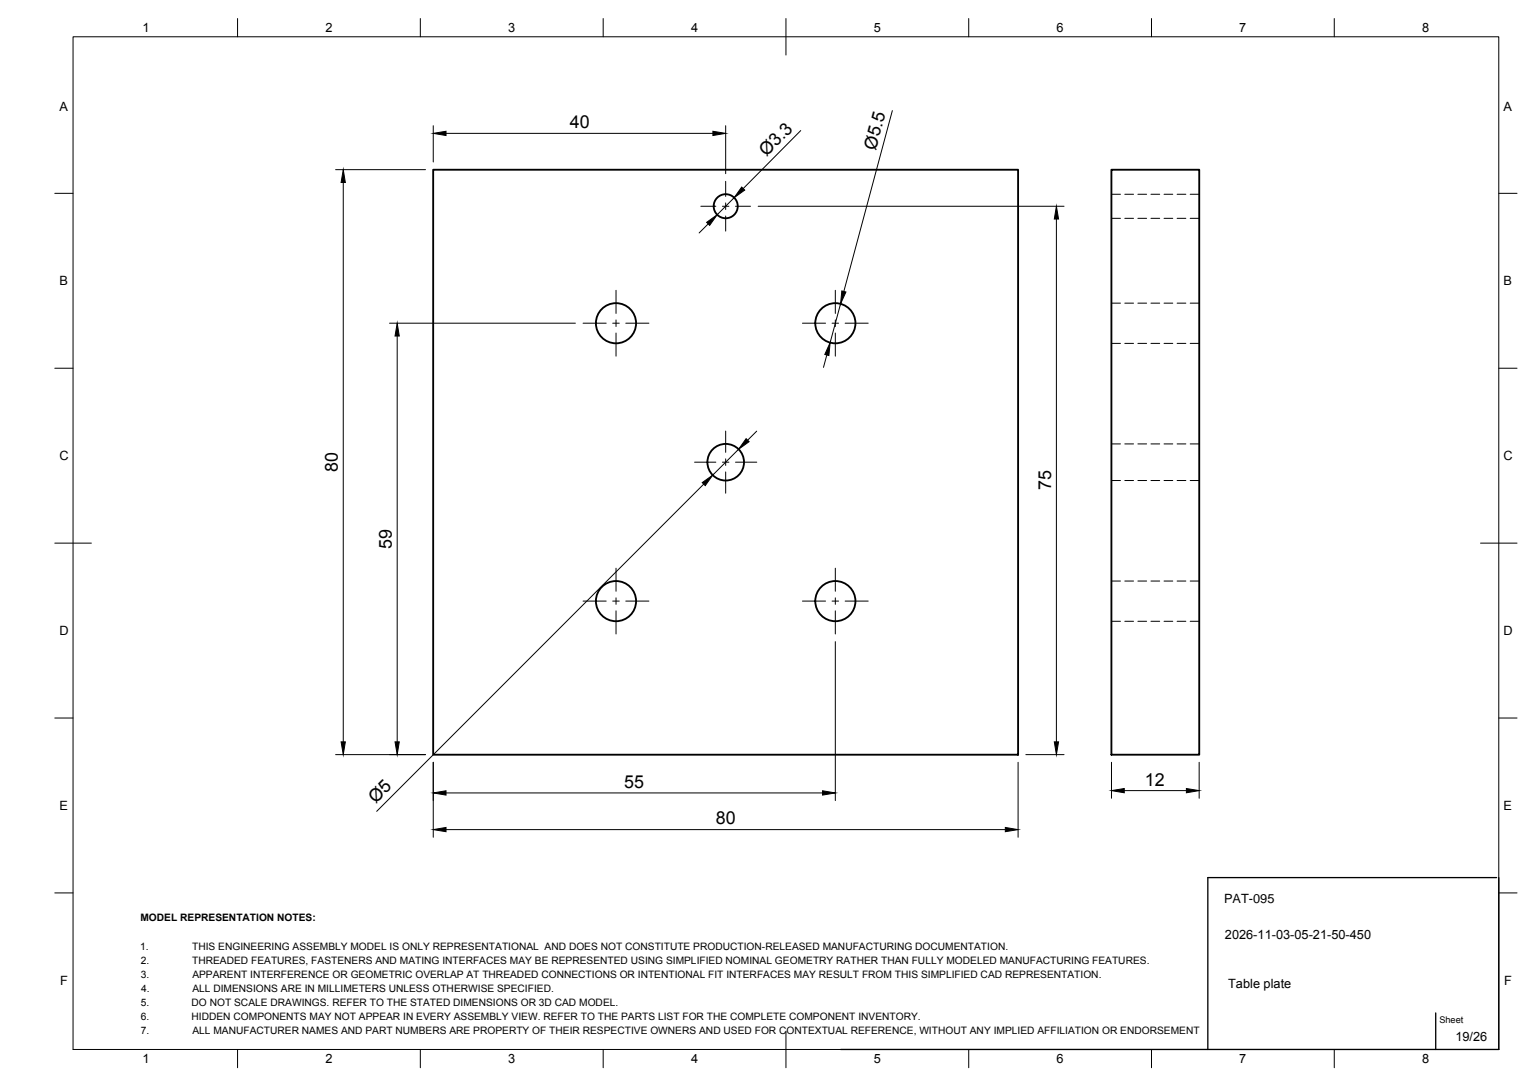
ISO-10303-21;
HEADER;
/* Generated by software containing ST-Developer
 * from STEP Tools, Inc. (www.steptools.com) 
 */

FILE_DESCRIPTION(
/* description */ ('Single-Axis Profile-Rail Linear Slide'),
/* implementation_level */ '2;1');

FILE_NAME(
/* name */ 'Table plate.step',
/* time_stamp */ '2026-10-27T10:47:43-07:00',
/* author */ (''),
/* organization */ (''),
/* preprocessor_version */ 'ST-DEVELOPER v20.2',
/* originating_system */ 'Autodesk Translation Framework v15.17.0.0',
/* authorisation */ '');

FILE_SCHEMA (('AUTOMOTIVE_DESIGN { 1 0 10303 214 3 1 1 }'));
ENDSEC;

DATA;
#10=MECHANICAL_DESIGN_GEOMETRIC_PRESENTATION_REPRESENTATION('',(#344),#14478);
#290=SHAPE_REPRESENTATION_RELATIONSHIP('SRR','None',#14621,#317);
#317=ADVANCED_BREP_SHAPE_REPRESENTATION('',(#369),#14465);
#344=STYLED_ITEM('',(#14824),#369);
#369=MANIFOLD_SOLID_BREP('Body1',#8606);
#439=FACE_BOUND('',#1690,.T.);
#440=FACE_BOUND('',#1691,.T.);
#441=FACE_BOUND('',#1692,.T.);
#442=FACE_BOUND('',#1693,.T.);
#443=FACE_BOUND('',#1694,.T.);
#444=FACE_BOUND('',#1695,.T.);
#445=FACE_BOUND('',#1697,.T.);
#446=FACE_BOUND('',#1698,.T.);
#447=FACE_BOUND('',#1699,.T.);
#448=FACE_BOUND('',#1700,.T.);
#449=FACE_BOUND('',#1701,.T.);
#450=FACE_BOUND('',#1702,.T.);
#747=PLANE('',#9365);
#748=PLANE('',#9366);
#749=PLANE('',#9367);
#750=PLANE('',#9368);
#751=PLANE('',#9369);
#752=PLANE('',#9370);
#1163=FACE_OUTER_BOUND('',#1679,.T.);
#1164=FACE_OUTER_BOUND('',#1680,.T.);
#1165=FACE_OUTER_BOUND('',#1681,.T.);
#1166=FACE_OUTER_BOUND('',#1682,.T.);
#1167=FACE_OUTER_BOUND('',#1683,.T.);
#1168=FACE_OUTER_BOUND('',#1684,.T.);
#1169=FACE_OUTER_BOUND('',#1685,.T.);
#1170=FACE_OUTER_BOUND('',#1686,.T.);
#1171=FACE_OUTER_BOUND('',#1687,.T.);
#1172=FACE_OUTER_BOUND('',#1688,.T.);
#1173=FACE_OUTER_BOUND('',#1689,.T.);
#1174=FACE_OUTER_BOUND('',#1696,.T.);
#1679=EDGE_LOOP('',(#7481,#7482,#7483,#7484));
#1680=EDGE_LOOP('',(#7485,#7486,#7487,#7488));
#1681=EDGE_LOOP('',(#7489,#7490,#7491,#7492));
#1682=EDGE_LOOP('',(#7493,#7494,#7495,#7496));
#1683=EDGE_LOOP('',(#7497,#7498,#7499,#7500));
#1684=EDGE_LOOP('',(#7501,#7502,#7503,#7504));
#1685=EDGE_LOOP('',(#7505,#7506,#7507,#7508));
#1686=EDGE_LOOP('',(#7509,#7510,#7511,#7512));
#1687=EDGE_LOOP('',(#7513,#7514,#7515,#7516));
#1688=EDGE_LOOP('',(#7517,#7518,#7519,#7520));
#1689=EDGE_LOOP('',(#7521,#7522,#7523,#7524));
#1690=EDGE_LOOP('',(#7525));
#1691=EDGE_LOOP('',(#7526));
#1692=EDGE_LOOP('',(#7527));
#1693=EDGE_LOOP('',(#7528));
#1694=EDGE_LOOP('',(#7529));
#1695=EDGE_LOOP('',(#7530));
#1696=EDGE_LOOP('',(#7531,#7532,#7533,#7534));
#1697=EDGE_LOOP('',(#7535));
#1698=EDGE_LOOP('',(#7536));
#1699=EDGE_LOOP('',(#7537));
#1700=EDGE_LOOP('',(#7538));
#1701=EDGE_LOOP('',(#7539));
#1702=EDGE_LOOP('',(#7540));
#2588=LINE('',#13730,#3559);
#2589=LINE('',#13736,#3560);
#2590=LINE('',#13742,#3561);
#2591=LINE('',#13748,#3562);
#2592=LINE('',#13754,#3563);
#2593=LINE('',#13760,#3564);
#2594=LINE('',#13765,#3565);
#2595=LINE('',#13767,#3566);
#2596=LINE('',#13769,#3567);
#2597=LINE('',#13770,#3568);
#2598=LINE('',#13773,#3569);
#2599=LINE('',#13775,#3570);
#2600=LINE('',#13776,#3571);
#2601=LINE('',#13779,#3572);
#2602=LINE('',#13781,#3573);
#2603=LINE('',#13782,#3574);
#2604=LINE('',#13784,#3575);
#2605=LINE('',#13785,#3576);
#3559=VECTOR('',#11229,0.164999999999999);
#3560=VECTOR('',#11236,0.25);
#3561=VECTOR('',#11243,0.275);
#3562=VECTOR('',#11250,0.275);
#3563=VECTOR('',#11257,0.275);
#3564=VECTOR('',#11264,0.275);
#3565=VECTOR('',#11269,1.);
#3566=VECTOR('',#11270,1.);
#3567=VECTOR('',#11271,1.);
#3568=VECTOR('',#11272,1.);
#3569=VECTOR('',#11275,1.);
#3570=VECTOR('',#11276,1.);
#3571=VECTOR('',#11277,1.);
#3572=VECTOR('',#11280,1.);
#3573=VECTOR('',#11281,1.);
#3574=VECTOR('',#11282,1.);
#3575=VECTOR('',#11285,1.);
#3576=VECTOR('',#11286,1.);
#3866=CIRCLE('',#9348,0.164999999999999);
#3867=CIRCLE('',#9349,0.164999999999999);
#3868=CIRCLE('',#9351,0.25);
#3869=CIRCLE('',#9352,0.25);
#3870=CIRCLE('',#9354,0.275);
#3871=CIRCLE('',#9355,0.275);
#3872=CIRCLE('',#9357,0.275);
#3873=CIRCLE('',#9358,0.275);
#3874=CIRCLE('',#9360,0.275);
#3875=CIRCLE('',#9361,0.275);
#3876=CIRCLE('',#9363,0.275);
#3877=CIRCLE('',#9364,0.275);
#4492=VERTEX_POINT('',#13727);
#4493=VERTEX_POINT('',#13729);
#4494=VERTEX_POINT('',#13733);
#4495=VERTEX_POINT('',#13735);
#4496=VERTEX_POINT('',#13739);
#4497=VERTEX_POINT('',#13741);
#4498=VERTEX_POINT('',#13745);
#4499=VERTEX_POINT('',#13747);
#4500=VERTEX_POINT('',#13751);
#4501=VERTEX_POINT('',#13753);
#4502=VERTEX_POINT('',#13757);
#4503=VERTEX_POINT('',#13759);
#4504=VERTEX_POINT('',#13763);
#4505=VERTEX_POINT('',#13764);
#4506=VERTEX_POINT('',#13766);
#4507=VERTEX_POINT('',#13768);
#4508=VERTEX_POINT('',#13772);
#4509=VERTEX_POINT('',#13774);
#4510=VERTEX_POINT('',#13778);
#4511=VERTEX_POINT('',#13780);
#5518=EDGE_CURVE('',#4492,#4492,#3866,.T.);
#5519=EDGE_CURVE('',#4492,#4493,#2588,.T.);
#5520=EDGE_CURVE('',#4493,#4493,#3867,.T.);
#5521=EDGE_CURVE('',#4494,#4494,#3868,.T.);
#5522=EDGE_CURVE('',#4494,#4495,#2589,.T.);
#5523=EDGE_CURVE('',#4495,#4495,#3869,.T.);
#5524=EDGE_CURVE('',#4496,#4496,#3870,.T.);
#5525=EDGE_CURVE('',#4496,#4497,#2590,.T.);
#5526=EDGE_CURVE('',#4497,#4497,#3871,.T.);
#5527=EDGE_CURVE('',#4498,#4498,#3872,.T.);
#5528=EDGE_CURVE('',#4498,#4499,#2591,.T.);
#5529=EDGE_CURVE('',#4499,#4499,#3873,.T.);
#5530=EDGE_CURVE('',#4500,#4500,#3874,.T.);
#5531=EDGE_CURVE('',#4500,#4501,#2592,.T.);
#5532=EDGE_CURVE('',#4501,#4501,#3875,.T.);
#5533=EDGE_CURVE('',#4502,#4502,#3876,.T.);
#5534=EDGE_CURVE('',#4502,#4503,#2593,.T.);
#5535=EDGE_CURVE('',#4503,#4503,#3877,.T.);
#5536=EDGE_CURVE('',#4504,#4505,#2594,.T.);
#5537=EDGE_CURVE('',#4505,#4506,#2595,.T.);
#5538=EDGE_CURVE('',#4507,#4506,#2596,.T.);
#5539=EDGE_CURVE('',#4504,#4507,#2597,.T.);
#5540=EDGE_CURVE('',#4508,#4504,#2598,.T.);
#5541=EDGE_CURVE('',#4509,#4507,#2599,.T.);
#5542=EDGE_CURVE('',#4508,#4509,#2600,.T.);
#5543=EDGE_CURVE('',#4510,#4508,#2601,.T.);
#5544=EDGE_CURVE('',#4511,#4509,#2602,.T.);
#5545=EDGE_CURVE('',#4510,#4511,#2603,.T.);
#5546=EDGE_CURVE('',#4505,#4510,#2604,.T.);
#5547=EDGE_CURVE('',#4506,#4511,#2605,.T.);
#7481=ORIENTED_EDGE('',*,*,#5518,.F.);
#7482=ORIENTED_EDGE('',*,*,#5519,.T.);
#7483=ORIENTED_EDGE('',*,*,#5520,.F.);
#7484=ORIENTED_EDGE('',*,*,#5519,.F.);
#7485=ORIENTED_EDGE('',*,*,#5521,.F.);
#7486=ORIENTED_EDGE('',*,*,#5522,.T.);
#7487=ORIENTED_EDGE('',*,*,#5523,.F.);
#7488=ORIENTED_EDGE('',*,*,#5522,.F.);
#7489=ORIENTED_EDGE('',*,*,#5524,.F.);
#7490=ORIENTED_EDGE('',*,*,#5525,.T.);
#7491=ORIENTED_EDGE('',*,*,#5526,.F.);
#7492=ORIENTED_EDGE('',*,*,#5525,.F.);
#7493=ORIENTED_EDGE('',*,*,#5527,.F.);
#7494=ORIENTED_EDGE('',*,*,#5528,.T.);
#7495=ORIENTED_EDGE('',*,*,#5529,.F.);
#7496=ORIENTED_EDGE('',*,*,#5528,.F.);
#7497=ORIENTED_EDGE('',*,*,#5530,.F.);
#7498=ORIENTED_EDGE('',*,*,#5531,.T.);
#7499=ORIENTED_EDGE('',*,*,#5532,.F.);
#7500=ORIENTED_EDGE('',*,*,#5531,.F.);
#7501=ORIENTED_EDGE('',*,*,#5533,.F.);
#7502=ORIENTED_EDGE('',*,*,#5534,.T.);
#7503=ORIENTED_EDGE('',*,*,#5535,.F.);
#7504=ORIENTED_EDGE('',*,*,#5534,.F.);
#7505=ORIENTED_EDGE('',*,*,#5536,.T.);
#7506=ORIENTED_EDGE('',*,*,#5537,.T.);
#7507=ORIENTED_EDGE('',*,*,#5538,.F.);
#7508=ORIENTED_EDGE('',*,*,#5539,.F.);
#7509=ORIENTED_EDGE('',*,*,#5540,.T.);
#7510=ORIENTED_EDGE('',*,*,#5539,.T.);
#7511=ORIENTED_EDGE('',*,*,#5541,.F.);
#7512=ORIENTED_EDGE('',*,*,#5542,.F.);
#7513=ORIENTED_EDGE('',*,*,#5543,.T.);
#7514=ORIENTED_EDGE('',*,*,#5542,.T.);
#7515=ORIENTED_EDGE('',*,*,#5544,.F.);
#7516=ORIENTED_EDGE('',*,*,#5545,.F.);
#7517=ORIENTED_EDGE('',*,*,#5546,.T.);
#7518=ORIENTED_EDGE('',*,*,#5545,.T.);
#7519=ORIENTED_EDGE('',*,*,#5547,.F.);
#7520=ORIENTED_EDGE('',*,*,#5537,.F.);
#7521=ORIENTED_EDGE('',*,*,#5547,.T.);
#7522=ORIENTED_EDGE('',*,*,#5544,.T.);
#7523=ORIENTED_EDGE('',*,*,#5541,.T.);
#7524=ORIENTED_EDGE('',*,*,#5538,.T.);
#7525=ORIENTED_EDGE('',*,*,#5520,.T.);
#7526=ORIENTED_EDGE('',*,*,#5523,.T.);
#7527=ORIENTED_EDGE('',*,*,#5526,.T.);
#7528=ORIENTED_EDGE('',*,*,#5529,.T.);
#7529=ORIENTED_EDGE('',*,*,#5532,.T.);
#7530=ORIENTED_EDGE('',*,*,#5535,.T.);
#7531=ORIENTED_EDGE('',*,*,#5546,.F.);
#7532=ORIENTED_EDGE('',*,*,#5536,.F.);
#7533=ORIENTED_EDGE('',*,*,#5540,.F.);
#7534=ORIENTED_EDGE('',*,*,#5543,.F.);
#7535=ORIENTED_EDGE('',*,*,#5518,.T.);
#7536=ORIENTED_EDGE('',*,*,#5521,.T.);
#7537=ORIENTED_EDGE('',*,*,#5524,.T.);
#7538=ORIENTED_EDGE('',*,*,#5527,.T.);
#7539=ORIENTED_EDGE('',*,*,#5530,.T.);
#7540=ORIENTED_EDGE('',*,*,#5533,.T.);
#8109=CYLINDRICAL_SURFACE('',#9347,0.164999999999999);
#8110=CYLINDRICAL_SURFACE('',#9350,0.25);
#8111=CYLINDRICAL_SURFACE('',#9353,0.275);
#8112=CYLINDRICAL_SURFACE('',#9356,0.275);
#8113=CYLINDRICAL_SURFACE('',#9359,0.275);
#8114=CYLINDRICAL_SURFACE('',#9362,0.275);
#8457=ADVANCED_FACE('',(#1163),#8109,.F.);
#8458=ADVANCED_FACE('',(#1164),#8110,.F.);
#8459=ADVANCED_FACE('',(#1165),#8111,.F.);
#8460=ADVANCED_FACE('',(#1166),#8112,.F.);
#8461=ADVANCED_FACE('',(#1167),#8113,.F.);
#8462=ADVANCED_FACE('',(#1168),#8114,.F.);
#8463=ADVANCED_FACE('',(#1169),#747,.T.);
#8464=ADVANCED_FACE('',(#1170),#748,.T.);
#8465=ADVANCED_FACE('',(#1171),#749,.T.);
#8466=ADVANCED_FACE('',(#1172),#750,.T.);
#8467=ADVANCED_FACE('',(#1173,#439,#440,#441,#442,#443,#444),#751,.T.);
#8468=ADVANCED_FACE('',(#1174,#445,#446,#447,#448,#449,#450),#752,.F.);
#8606=CLOSED_SHELL('',(#8457,#8458,#8459,#8460,#8461,#8462,#8463,#8464,
#8465,#8466,#8467,#8468));
#9346=AXIS2_PLACEMENT_3D('',#13725,#11223,#11224);
#9347=AXIS2_PLACEMENT_3D('',#13726,#11225,#11226);
#9348=AXIS2_PLACEMENT_3D('',#13728,#11227,#11228);
#9349=AXIS2_PLACEMENT_3D('',#13731,#11230,#11231);
#9350=AXIS2_PLACEMENT_3D('',#13732,#11232,#11233);
#9351=AXIS2_PLACEMENT_3D('',#13734,#11234,#11235);
#9352=AXIS2_PLACEMENT_3D('',#13737,#11237,#11238);
#9353=AXIS2_PLACEMENT_3D('',#13738,#11239,#11240);
#9354=AXIS2_PLACEMENT_3D('',#13740,#11241,#11242);
#9355=AXIS2_PLACEMENT_3D('',#13743,#11244,#11245);
#9356=AXIS2_PLACEMENT_3D('',#13744,#11246,#11247);
#9357=AXIS2_PLACEMENT_3D('',#13746,#11248,#11249);
#9358=AXIS2_PLACEMENT_3D('',#13749,#11251,#11252);
#9359=AXIS2_PLACEMENT_3D('',#13750,#11253,#11254);
#9360=AXIS2_PLACEMENT_3D('',#13752,#11255,#11256);
#9361=AXIS2_PLACEMENT_3D('',#13755,#11258,#11259);
#9362=AXIS2_PLACEMENT_3D('',#13756,#11260,#11261);
#9363=AXIS2_PLACEMENT_3D('',#13758,#11262,#11263);
#9364=AXIS2_PLACEMENT_3D('',#13761,#11265,#11266);
#9365=AXIS2_PLACEMENT_3D('',#13762,#11267,#11268);
#9366=AXIS2_PLACEMENT_3D('',#13771,#11273,#11274);
#9367=AXIS2_PLACEMENT_3D('',#13777,#11278,#11279);
#9368=AXIS2_PLACEMENT_3D('',#13783,#11283,#11284);
#9369=AXIS2_PLACEMENT_3D('',#13786,#11287,#11288);
#9370=AXIS2_PLACEMENT_3D('',#13787,#11289,#11290);
#11223=DIRECTION('axis',(0.,0.,1.));
#11224=DIRECTION('refdir',(1.,0.,0.));
#11225=DIRECTION('center_axis',(0.,0.,1.));
#11226=DIRECTION('ref_axis',(1.,0.,0.));
#11227=DIRECTION('center_axis',(0.,0.,1.));
#11228=DIRECTION('ref_axis',(1.,0.,0.));
#11229=DIRECTION('',(0.,0.,1.));
#11230=DIRECTION('center_axis',(0.,0.,-1.));
#11231=DIRECTION('ref_axis',(1.,0.,0.));
#11232=DIRECTION('center_axis',(0.,0.,1.));
#11233=DIRECTION('ref_axis',(1.,0.,0.));
#11234=DIRECTION('center_axis',(0.,0.,1.));
#11235=DIRECTION('ref_axis',(1.,0.,0.));
#11236=DIRECTION('',(0.,0.,1.));
#11237=DIRECTION('center_axis',(0.,0.,-1.));
#11238=DIRECTION('ref_axis',(1.,0.,0.));
#11239=DIRECTION('center_axis',(0.,0.,1.));
#11240=DIRECTION('ref_axis',(1.,0.,0.));
#11241=DIRECTION('center_axis',(0.,0.,1.));
#11242=DIRECTION('ref_axis',(1.,0.,0.));
#11243=DIRECTION('',(0.,0.,1.));
#11244=DIRECTION('center_axis',(0.,0.,-1.));
#11245=DIRECTION('ref_axis',(1.,0.,0.));
#11246=DIRECTION('center_axis',(0.,0.,1.));
#11247=DIRECTION('ref_axis',(1.,0.,0.));
#11248=DIRECTION('center_axis',(0.,0.,1.));
#11249=DIRECTION('ref_axis',(1.,0.,0.));
#11250=DIRECTION('',(0.,0.,1.));
#11251=DIRECTION('center_axis',(0.,0.,-1.));
#11252=DIRECTION('ref_axis',(1.,0.,0.));
#11253=DIRECTION('center_axis',(0.,0.,1.));
#11254=DIRECTION('ref_axis',(1.,0.,0.));
#11255=DIRECTION('center_axis',(0.,0.,1.));
#11256=DIRECTION('ref_axis',(1.,0.,0.));
#11257=DIRECTION('',(0.,0.,1.));
#11258=DIRECTION('center_axis',(0.,0.,-1.));
#11259=DIRECTION('ref_axis',(1.,0.,0.));
#11260=DIRECTION('center_axis',(0.,0.,1.));
#11261=DIRECTION('ref_axis',(1.,0.,0.));
#11262=DIRECTION('center_axis',(0.,0.,1.));
#11263=DIRECTION('ref_axis',(1.,0.,0.));
#11264=DIRECTION('',(0.,0.,1.));
#11265=DIRECTION('center_axis',(0.,0.,-1.));
#11266=DIRECTION('ref_axis',(1.,0.,0.));
#11267=DIRECTION('center_axis',(0.,1.,0.));
#11268=DIRECTION('ref_axis',(-1.,0.,0.));
#11269=DIRECTION('',(-1.,0.,0.));
#11270=DIRECTION('',(0.,0.,1.));
#11271=DIRECTION('',(-1.,0.,0.));
#11272=DIRECTION('',(0.,0.,1.));
#11273=DIRECTION('center_axis',(1.,0.,0.));
#11274=DIRECTION('ref_axis',(0.,1.,0.));
#11275=DIRECTION('',(0.,1.,0.));
#11276=DIRECTION('',(0.,1.,0.));
#11277=DIRECTION('',(0.,0.,1.));
#11278=DIRECTION('center_axis',(0.,-1.,0.));
#11279=DIRECTION('ref_axis',(1.,0.,0.));
#11280=DIRECTION('',(1.,0.,0.));
#11281=DIRECTION('',(1.,0.,0.));
#11282=DIRECTION('',(0.,0.,1.));
#11283=DIRECTION('center_axis',(-1.,0.,0.));
#11284=DIRECTION('ref_axis',(0.,-1.,0.));
#11285=DIRECTION('',(0.,-1.,0.));
#11286=DIRECTION('',(0.,-1.,0.));
#11287=DIRECTION('center_axis',(0.,0.,1.));
#11288=DIRECTION('ref_axis',(1.,0.,0.));
#11289=DIRECTION('center_axis',(0.,0.,1.));
#11290=DIRECTION('ref_axis',(1.,0.,0.));
#13725=CARTESIAN_POINT('',(0.,0.,0.));
#13726=CARTESIAN_POINT('Origin',(11.,3.5,5.1));
#13727=CARTESIAN_POINT('',(10.835,3.5,5.2));
#13728=CARTESIAN_POINT('Origin',(11.,3.5,5.2));
#13729=CARTESIAN_POINT('',(10.835,3.5,6.4));
#13730=CARTESIAN_POINT('',(10.835,3.5,5.1));
#13731=CARTESIAN_POINT('Origin',(11.,3.5,6.4));
#13732=CARTESIAN_POINT('Origin',(11.,0.,5.1));
#13733=CARTESIAN_POINT('',(10.75,-3.06161699786838E-17,5.2));
#13734=CARTESIAN_POINT('Origin',(11.,0.,5.2));
#13735=CARTESIAN_POINT('',(10.75,3.06161699786838E-17,6.4));
#13736=CARTESIAN_POINT('',(10.75,-3.06161699786838E-17,5.1));
#13737=CARTESIAN_POINT('Origin',(11.,0.,6.4));
#13738=CARTESIAN_POINT('Origin',(12.5,-1.9,5.1));
#13739=CARTESIAN_POINT('',(12.225,-1.9,5.2));
#13740=CARTESIAN_POINT('Origin',(12.5,-1.9,5.2));
#13741=CARTESIAN_POINT('',(12.225,-1.9,6.4));
#13742=CARTESIAN_POINT('',(12.225,-1.9,5.1));
#13743=CARTESIAN_POINT('Origin',(12.5,-1.9,6.4));
#13744=CARTESIAN_POINT('Origin',(9.5,1.9,5.1));
#13745=CARTESIAN_POINT('',(9.225,1.9,5.2));
#13746=CARTESIAN_POINT('Origin',(9.5,1.9,5.2));
#13747=CARTESIAN_POINT('',(9.225,1.9,6.4));
#13748=CARTESIAN_POINT('',(9.225,1.9,5.1));
#13749=CARTESIAN_POINT('Origin',(9.5,1.9,6.4));
#13750=CARTESIAN_POINT('Origin',(9.5,-1.9,5.1));
#13751=CARTESIAN_POINT('',(9.225,-1.9,5.2));
#13752=CARTESIAN_POINT('Origin',(9.5,-1.9,5.2));
#13753=CARTESIAN_POINT('',(9.225,-1.9,6.4));
#13754=CARTESIAN_POINT('',(9.225,-1.9,5.1));
#13755=CARTESIAN_POINT('Origin',(9.5,-1.9,6.4));
#13756=CARTESIAN_POINT('Origin',(12.5,1.9,5.1));
#13757=CARTESIAN_POINT('',(12.225,1.9,5.2));
#13758=CARTESIAN_POINT('Origin',(12.5,1.9,5.2));
#13759=CARTESIAN_POINT('',(12.225,1.9,6.4));
#13760=CARTESIAN_POINT('',(12.225,1.9,5.1));
#13761=CARTESIAN_POINT('Origin',(12.5,1.9,6.4));
#13762=CARTESIAN_POINT('Origin',(15.,4.,5.2));
#13763=CARTESIAN_POINT('',(15.,4.,5.2));
#13764=CARTESIAN_POINT('',(7.,4.,5.2));
#13765=CARTESIAN_POINT('',(15.,4.,5.2));
#13766=CARTESIAN_POINT('',(7.,4.,6.4));
#13767=CARTESIAN_POINT('',(7.,4.,5.2));
#13768=CARTESIAN_POINT('',(15.,4.,6.4));
#13769=CARTESIAN_POINT('',(15.,4.,6.4));
#13770=CARTESIAN_POINT('',(15.,4.,5.2));
#13771=CARTESIAN_POINT('Origin',(15.,-4.,5.2));
#13772=CARTESIAN_POINT('',(15.,-4.,5.2));
#13773=CARTESIAN_POINT('',(15.,-4.,5.2));
#13774=CARTESIAN_POINT('',(15.,-4.,6.4));
#13775=CARTESIAN_POINT('',(15.,-4.,6.4));
#13776=CARTESIAN_POINT('',(15.,-4.,5.2));
#13777=CARTESIAN_POINT('Origin',(7.,-4.,5.2));
#13778=CARTESIAN_POINT('',(7.,-4.,5.2));
#13779=CARTESIAN_POINT('',(7.,-4.,5.2));
#13780=CARTESIAN_POINT('',(7.,-4.,6.4));
#13781=CARTESIAN_POINT('',(7.,-4.,6.4));
#13782=CARTESIAN_POINT('',(7.,-4.,5.2));
#13783=CARTESIAN_POINT('Origin',(7.,4.,5.2));
#13784=CARTESIAN_POINT('',(7.,4.,5.2));
#13785=CARTESIAN_POINT('',(7.,4.,6.4));
#13786=CARTESIAN_POINT('Origin',(11.,0.,6.4));
#13787=CARTESIAN_POINT('Origin',(11.,0.,5.2));
#14433=UNCERTAINTY_MEASURE_WITH_UNIT(LENGTH_MEASURE(0.001),#14479,
'DISTANCE_ACCURACY_VALUE',
'Maximum model space distance between geometric entities at asserted c
onnectivities');
#14446=UNCERTAINTY_MEASURE_WITH_UNIT(LENGTH_MEASURE(0.001),#14479,
'DISTANCE_ACCURACY_VALUE',
'Maximum model space distance between geometric entities at asserted c
onnectivities');
#14465=(
GEOMETRIC_REPRESENTATION_CONTEXT(3)
GLOBAL_UNCERTAINTY_ASSIGNED_CONTEXT((#14433))
GLOBAL_UNIT_ASSIGNED_CONTEXT((#14479,#14481,#14482))
REPRESENTATION_CONTEXT('','3D')
);
#14478=(
GEOMETRIC_REPRESENTATION_CONTEXT(3)
GLOBAL_UNCERTAINTY_ASSIGNED_CONTEXT((#14446))
GLOBAL_UNIT_ASSIGNED_CONTEXT((#14479,#14481,#14482))
REPRESENTATION_CONTEXT('','3D')
);
#14479=(
LENGTH_UNIT()
NAMED_UNIT(*)
SI_UNIT(.CENTI.,.METRE.)
);
#14481=(
NAMED_UNIT(*)
PLANE_ANGLE_UNIT()
SI_UNIT($,.RADIAN.)
);
#14482=(
NAMED_UNIT(*)
SI_UNIT($,.STERADIAN.)
SOLID_ANGLE_UNIT()
);
#14501=SHAPE_DEFINITION_REPRESENTATION(#14532,#14621);
#14532=PRODUCT_DEFINITION_SHAPE('',$,#14653);
#14621=SHAPE_REPRESENTATION('',(#9346),#14465);
#14634=PRODUCT_DEFINITION_CONTEXT('part definition',#14729,'design');
#14653=PRODUCT_DEFINITION('Table plate','Table plate',#14684,#14634);
#14684=PRODUCT_DEFINITION_FORMATION('',$,#14749);
#14729=APPLICATION_CONTEXT(
'Core Data for Automotive Mechanical Design Process');
#14730=PRODUCT_CONTEXT('part definition',#14729,'mechanical');
#14749=PRODUCT('Table plate','Table plate','Table plate',(#14730));
#14818=COLOUR_RGB('Sky Blue',0.24,0.69,0.87);
#14819=FILL_AREA_STYLE_COLOUR('',#14818);
#14820=FILL_AREA_STYLE('',(#14819));
#14821=SURFACE_STYLE_FILL_AREA(#14820);
#14822=SURFACE_SIDE_STYLE('',(#14821));
#14823=SURFACE_STYLE_USAGE(.BOTH.,#14822);
#14824=PRESENTATION_STYLE_ASSIGNMENT((#14823));
ENDSEC;
END-ISO-10303-21;
